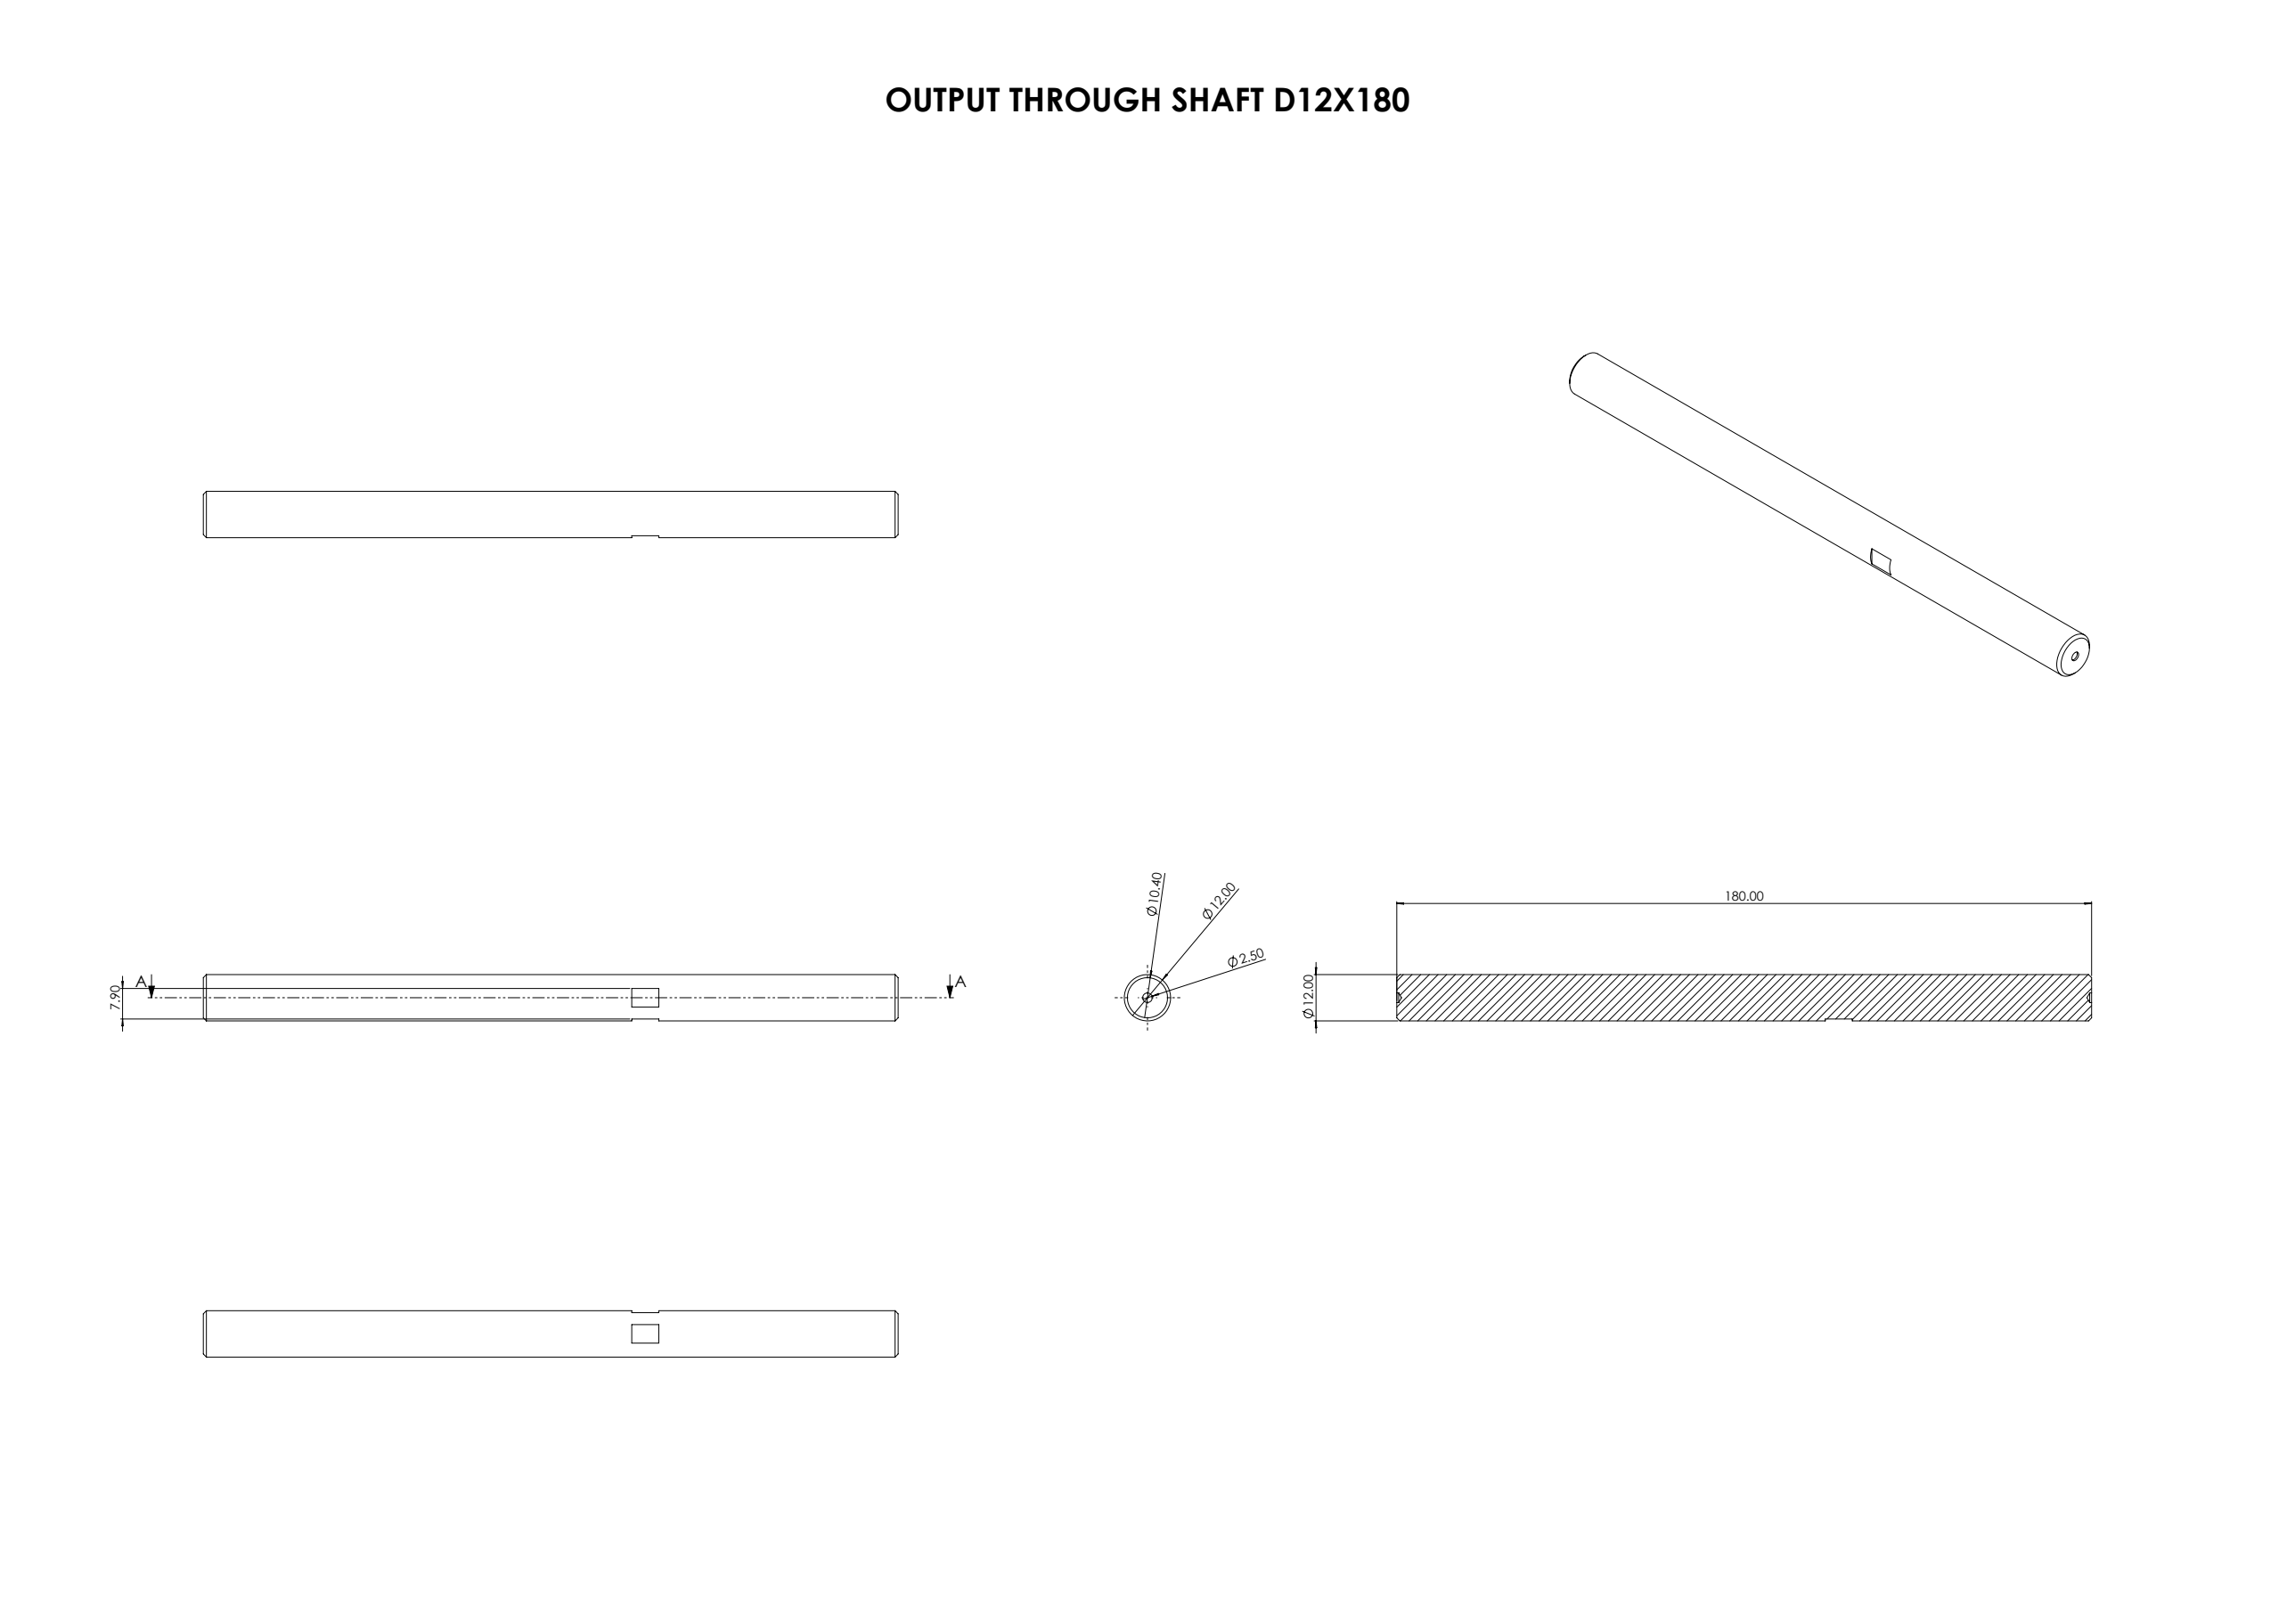
ISO-10303-21;
HEADER;
/* Generated by software containing ST-Developer
 * from STEP Tools, Inc. (www.steptools.com) 
 */

FILE_DESCRIPTION(
/* description */ (''),
/* implementation_level */ '2;1');

FILE_NAME(
/* name */ '05_Output_Through_Shaft_D12x180.step',
/* time_stamp */ '2026-10-11T09:12:28-07:00',
/* author */ (''),
/* organization */ (''),
/* preprocessor_version */ 'ST-DEVELOPER v20.2',
/* originating_system */ 'Autodesk Translation Framework v15.15.0.0',
/* authorisation */ '');

FILE_SCHEMA (('AUTOMOTIVE_DESIGN { 1 0 10303 214 3 1 1 }'));
ENDSEC;

DATA;
#10=MECHANICAL_DESIGN_GEOMETRIC_PRESENTATION_REPRESENTATION('',(#651),#23254);
#631=SHAPE_REPRESENTATION_RELATIONSHIP('SRR','None',#23304,#641);
#641=ADVANCED_BREP_SHAPE_REPRESENTATION('',(#661),#23248);
#651=STYLED_ITEM('',(#23462),#661);
#661=MANIFOLD_SOLID_BREP('Body1',#7029);
#739=CONICAL_SURFACE('',#7587,0.625,1.04746029293308);
#740=CONICAL_SURFACE('',#7594,1.25,1.04746029293308);
#741=CONICAL_SURFACE('',#7597,5.6,0.785398163397448);
#742=CONICAL_SURFACE('',#7601,5.6,0.785398163397448);
#811=FACE_BOUND('',#1692,.T.);
#812=FACE_BOUND('',#1695,.T.);
#813=FACE_BOUND('',#1698,.T.);
#940=PLANE('',#7575);
#941=PLANE('',#7578);
#942=PLANE('',#7581);
#943=PLANE('',#7582);
#944=PLANE('',#7584);
#945=PLANE('',#7585);
#946=PLANE('',#7595);
#947=PLANE('',#7603);
#1255=FACE_OUTER_BOUND('',#1681,.T.);
#1256=FACE_OUTER_BOUND('',#1682,.T.);
#1257=FACE_OUTER_BOUND('',#1683,.T.);
#1258=FACE_OUTER_BOUND('',#1684,.T.);
#1259=FACE_OUTER_BOUND('',#1685,.T.);
#1260=FACE_OUTER_BOUND('',#1686,.T.);
#1261=FACE_OUTER_BOUND('',#1687,.T.);
#1262=FACE_OUTER_BOUND('',#1688,.T.);
#1263=FACE_OUTER_BOUND('',#1689,.T.);
#1264=FACE_OUTER_BOUND('',#1690,.T.);
#1265=FACE_OUTER_BOUND('',#1691,.T.);
#1266=FACE_OUTER_BOUND('',#1693,.T.);
#1267=FACE_OUTER_BOUND('',#1694,.T.);
#1268=FACE_OUTER_BOUND('',#1696,.T.);
#1269=FACE_OUTER_BOUND('',#1697,.T.);
#1681=EDGE_LOOP('',(#5933,#5934,#5935));
#1682=EDGE_LOOP('',(#5936,#5937,#5938));
#1683=EDGE_LOOP('',(#5939,#5940,#5941,#5942));
#1684=EDGE_LOOP('',(#5943,#5944));
#1685=EDGE_LOOP('',(#5945,#5946,#5947,#5948));
#1686=EDGE_LOOP('',(#5949,#5950));
#1687=EDGE_LOOP('',(#5951,#5952,#5953));
#1688=EDGE_LOOP('',(#5954,#5955,#5956,#5957));
#1689=EDGE_LOOP('',(#5958,#5959,#5960,#5961));
#1690=EDGE_LOOP('',(#5962,#5963,#5964));
#1691=EDGE_LOOP('',(#5965));
#1692=EDGE_LOOP('',(#5966));
#1693=EDGE_LOOP('',(#5967,#5968,#5969,#5970));
#1694=EDGE_LOOP('',(#5971,#5972,#5973,#5974,#5975,#5976,#5977,#5978,#5979,
#5980,#5981,#5982));
#1695=EDGE_LOOP('',(#5983,#5984,#5985,#5986));
#1696=EDGE_LOOP('',(#5987,#5988,#5989,#5990));
#1697=EDGE_LOOP('',(#5991));
#1698=EDGE_LOOP('',(#5992));
#2009=LINE('',#21048,#2268);
#2010=LINE('',#21055,#2269);
#2011=LINE('',#21058,#2270);
#2012=LINE('',#21059,#2271);
#2013=LINE('',#21064,#2272);
#2014=LINE('',#21067,#2273);
#2015=LINE('',#21069,#2274);
#2016=LINE('',#21070,#2275);
#2017=LINE('',#21076,#2276);
#2018=LINE('',#21080,#2277);
#2019=LINE('',#21086,#2278);
#2020=LINE('',#21090,#2279);
#2021=LINE('',#21097,#2280);
#2022=LINE('',#21101,#2281);
#2023=LINE('',#21102,#2282);
#2024=LINE('',#21106,#2283);
#2268=VECTOR('',#8861,10.);
#2269=VECTOR('',#8868,10.);
#2270=VECTOR('',#8873,10.);
#2271=VECTOR('',#8874,10.);
#2272=VECTOR('',#8879,10.);
#2273=VECTOR('',#8882,10.);
#2274=VECTOR('',#8883,10.);
#2275=VECTOR('',#8884,10.);
#2276=VECTOR('',#8891,0.625);
#2277=VECTOR('',#8896,1.25);
#2278=VECTOR('',#8903,1.25);
#2279=VECTOR('',#8908,1.25);
#2280=VECTOR('',#8917,5.6);
#2281=VECTOR('',#8922,6.);
#2282=VECTOR('',#8923,6.);
#2283=VECTOR('',#8928,5.6);
#2586=CIRCLE('',#7576,6.);
#2587=CIRCLE('',#7577,6.);
#2588=CIRCLE('',#7579,6.);
#2589=CIRCLE('',#7580,6.);
#2590=CIRCLE('',#7583,6.);
#2591=CIRCLE('',#7586,6.);
#2592=CIRCLE('',#7588,1.25);
#2593=CIRCLE('',#7590,1.25);
#2594=CIRCLE('',#7592,1.25);
#2595=CIRCLE('',#7593,1.25);
#2596=CIRCLE('',#7596,5.2);
#2597=CIRCLE('',#7598,6.);
#2598=CIRCLE('',#7600,6.);
#2599=CIRCLE('',#7602,5.2);
#3184=VERTEX_POINT('',#21044);
#3185=VERTEX_POINT('',#21045);
#3186=VERTEX_POINT('',#21047);
#3187=VERTEX_POINT('',#21051);
#3188=VERTEX_POINT('',#21052);
#3189=VERTEX_POINT('',#21054);
#3190=VERTEX_POINT('',#21061);
#3191=VERTEX_POINT('',#21062);
#3192=VERTEX_POINT('',#21066);
#3193=VERTEX_POINT('',#21068);
#3194=VERTEX_POINT('',#21074);
#3195=VERTEX_POINT('',#21075);
#3196=VERTEX_POINT('',#21079);
#3197=VERTEX_POINT('',#21083);
#3198=VERTEX_POINT('',#21085);
#3199=VERTEX_POINT('',#21089);
#3200=VERTEX_POINT('',#21092);
#3201=VERTEX_POINT('',#21095);
#3202=VERTEX_POINT('',#21099);
#3203=VERTEX_POINT('',#21104);
#4142=EDGE_CURVE('',#3184,#3185,#2586,.T.);
#4143=EDGE_CURVE('',#3184,#3186,#2009,.T.);
#4144=EDGE_CURVE('',#3185,#3186,#2587,.T.);
#4145=EDGE_CURVE('',#3187,#3188,#2588,.T.);
#4146=EDGE_CURVE('',#3187,#3189,#2010,.T.);
#4147=EDGE_CURVE('',#3188,#3189,#2589,.T.);
#4148=EDGE_CURVE('',#3189,#3184,#2011,.T.);
#4149=EDGE_CURVE('',#3186,#3187,#2012,.T.);
#4150=EDGE_CURVE('',#3190,#3191,#2590,.T.);
#4151=EDGE_CURVE('',#3190,#3191,#2013,.T.);
#4152=EDGE_CURVE('',#3192,#3190,#2014,.T.);
#4153=EDGE_CURVE('',#3193,#3192,#2015,.T.);
#4154=EDGE_CURVE('',#3191,#3193,#2016,.T.);
#4155=EDGE_CURVE('',#3193,#3192,#2591,.T.);
#4156=EDGE_CURVE('',#3194,#3195,#2017,.T.);
#4157=EDGE_CURVE('',#3195,#3195,#2592,.T.);
#4158=EDGE_CURVE('',#3195,#3196,#2018,.T.);
#4159=EDGE_CURVE('',#3196,#3196,#2593,.T.);
#4160=EDGE_CURVE('',#3197,#3197,#2594,.T.);
#4161=EDGE_CURVE('',#3197,#3198,#2019,.T.);
#4162=EDGE_CURVE('',#3198,#3198,#2595,.T.);
#4163=EDGE_CURVE('',#3198,#3199,#2020,.T.);
#4164=EDGE_CURVE('',#3200,#3200,#2596,.T.);
#4165=EDGE_CURVE('',#3201,#3201,#2597,.T.);
#4166=EDGE_CURVE('',#3201,#3200,#2021,.T.);
#4167=EDGE_CURVE('',#3202,#3202,#2598,.T.);
#4168=EDGE_CURVE('',#3202,#3188,#2022,.T.);
#4169=EDGE_CURVE('',#3185,#3201,#2023,.T.);
#4170=EDGE_CURVE('',#3203,#3203,#2599,.T.);
#4171=EDGE_CURVE('',#3203,#3202,#2024,.T.);
#5933=ORIENTED_EDGE('',*,*,#4142,.F.);
#5934=ORIENTED_EDGE('',*,*,#4143,.T.);
#5935=ORIENTED_EDGE('',*,*,#4144,.F.);
#5936=ORIENTED_EDGE('',*,*,#4145,.F.);
#5937=ORIENTED_EDGE('',*,*,#4146,.T.);
#5938=ORIENTED_EDGE('',*,*,#4147,.F.);
#5939=ORIENTED_EDGE('',*,*,#4148,.F.);
#5940=ORIENTED_EDGE('',*,*,#4146,.F.);
#5941=ORIENTED_EDGE('',*,*,#4149,.F.);
#5942=ORIENTED_EDGE('',*,*,#4143,.F.);
#5943=ORIENTED_EDGE('',*,*,#4150,.F.);
#5944=ORIENTED_EDGE('',*,*,#4151,.T.);
#5945=ORIENTED_EDGE('',*,*,#4152,.F.);
#5946=ORIENTED_EDGE('',*,*,#4153,.F.);
#5947=ORIENTED_EDGE('',*,*,#4154,.F.);
#5948=ORIENTED_EDGE('',*,*,#4151,.F.);
#5949=ORIENTED_EDGE('',*,*,#4155,.F.);
#5950=ORIENTED_EDGE('',*,*,#4153,.T.);
#5951=ORIENTED_EDGE('',*,*,#4156,.T.);
#5952=ORIENTED_EDGE('',*,*,#4157,.T.);
#5953=ORIENTED_EDGE('',*,*,#4156,.F.);
#5954=ORIENTED_EDGE('',*,*,#4157,.F.);
#5955=ORIENTED_EDGE('',*,*,#4158,.T.);
#5956=ORIENTED_EDGE('',*,*,#4159,.F.);
#5957=ORIENTED_EDGE('',*,*,#4158,.F.);
#5958=ORIENTED_EDGE('',*,*,#4160,.F.);
#5959=ORIENTED_EDGE('',*,*,#4161,.T.);
#5960=ORIENTED_EDGE('',*,*,#4162,.T.);
#5961=ORIENTED_EDGE('',*,*,#4161,.F.);
#5962=ORIENTED_EDGE('',*,*,#4162,.F.);
#5963=ORIENTED_EDGE('',*,*,#4163,.T.);
#5964=ORIENTED_EDGE('',*,*,#4163,.F.);
#5965=ORIENTED_EDGE('',*,*,#4164,.F.);
#5966=ORIENTED_EDGE('',*,*,#4160,.T.);
#5967=ORIENTED_EDGE('',*,*,#4165,.F.);
#5968=ORIENTED_EDGE('',*,*,#4166,.T.);
#5969=ORIENTED_EDGE('',*,*,#4164,.T.);
#5970=ORIENTED_EDGE('',*,*,#4166,.F.);
#5971=ORIENTED_EDGE('',*,*,#4167,.F.);
#5972=ORIENTED_EDGE('',*,*,#4168,.T.);
#5973=ORIENTED_EDGE('',*,*,#4147,.T.);
#5974=ORIENTED_EDGE('',*,*,#4148,.T.);
#5975=ORIENTED_EDGE('',*,*,#4142,.T.);
#5976=ORIENTED_EDGE('',*,*,#4169,.T.);
#5977=ORIENTED_EDGE('',*,*,#4165,.T.);
#5978=ORIENTED_EDGE('',*,*,#4169,.F.);
#5979=ORIENTED_EDGE('',*,*,#4144,.T.);
#5980=ORIENTED_EDGE('',*,*,#4149,.T.);
#5981=ORIENTED_EDGE('',*,*,#4145,.T.);
#5982=ORIENTED_EDGE('',*,*,#4168,.F.);
#5983=ORIENTED_EDGE('',*,*,#4154,.T.);
#5984=ORIENTED_EDGE('',*,*,#4155,.T.);
#5985=ORIENTED_EDGE('',*,*,#4152,.T.);
#5986=ORIENTED_EDGE('',*,*,#4150,.T.);
#5987=ORIENTED_EDGE('',*,*,#4170,.F.);
#5988=ORIENTED_EDGE('',*,*,#4171,.T.);
#5989=ORIENTED_EDGE('',*,*,#4167,.T.);
#5990=ORIENTED_EDGE('',*,*,#4171,.F.);
#5991=ORIENTED_EDGE('',*,*,#4170,.T.);
#5992=ORIENTED_EDGE('',*,*,#4159,.T.);
#6602=CYLINDRICAL_SURFACE('',#7589,1.25);
#6603=CYLINDRICAL_SURFACE('',#7591,1.25);
#6604=CYLINDRICAL_SURFACE('',#7599,6.);
#6906=ADVANCED_FACE('',(#1255),#940,.F.);
#6907=ADVANCED_FACE('',(#1256),#941,.F.);
#6908=ADVANCED_FACE('',(#1257),#942,.F.);
#6909=ADVANCED_FACE('',(#1258),#943,.F.);
#6910=ADVANCED_FACE('',(#1259),#944,.F.);
#6911=ADVANCED_FACE('',(#1260),#945,.F.);
#6912=ADVANCED_FACE('',(#1261),#739,.F.);
#6913=ADVANCED_FACE('',(#1262),#6602,.F.);
#6914=ADVANCED_FACE('',(#1263),#6603,.F.);
#6915=ADVANCED_FACE('',(#1264),#740,.F.);
#6916=ADVANCED_FACE('',(#1265,#811),#946,.T.);
#6917=ADVANCED_FACE('',(#1266),#741,.T.);
#6918=ADVANCED_FACE('',(#1267,#812),#6604,.T.);
#6919=ADVANCED_FACE('',(#1268),#742,.T.);
#6920=ADVANCED_FACE('',(#1269,#813),#947,.T.);
#7029=CLOSED_SHELL('',(#6906,#6907,#6908,#6909,#6910,#6911,#6912,#6913,
#6914,#6915,#6916,#6917,#6918,#6919,#6920));
#7574=AXIS2_PLACEMENT_3D('',#21042,#8855,#8856);
#7575=AXIS2_PLACEMENT_3D('',#21043,#8857,#8858);
#7576=AXIS2_PLACEMENT_3D('',#21046,#8859,#8860);
#7577=AXIS2_PLACEMENT_3D('',#21049,#8862,#8863);
#7578=AXIS2_PLACEMENT_3D('',#21050,#8864,#8865);
#7579=AXIS2_PLACEMENT_3D('',#21053,#8866,#8867);
#7580=AXIS2_PLACEMENT_3D('',#21056,#8869,#8870);
#7581=AXIS2_PLACEMENT_3D('',#21057,#8871,#8872);
#7582=AXIS2_PLACEMENT_3D('',#21060,#8875,#8876);
#7583=AXIS2_PLACEMENT_3D('',#21063,#8877,#8878);
#7584=AXIS2_PLACEMENT_3D('',#21065,#8880,#8881);
#7585=AXIS2_PLACEMENT_3D('',#21071,#8885,#8886);
#7586=AXIS2_PLACEMENT_3D('',#21072,#8887,#8888);
#7587=AXIS2_PLACEMENT_3D('',#21073,#8889,#8890);
#7588=AXIS2_PLACEMENT_3D('',#21077,#8892,#8893);
#7589=AXIS2_PLACEMENT_3D('',#21078,#8894,#8895);
#7590=AXIS2_PLACEMENT_3D('',#21081,#8897,#8898);
#7591=AXIS2_PLACEMENT_3D('',#21082,#8899,#8900);
#7592=AXIS2_PLACEMENT_3D('',#21084,#8901,#8902);
#7593=AXIS2_PLACEMENT_3D('',#21087,#8904,#8905);
#7594=AXIS2_PLACEMENT_3D('',#21088,#8906,#8907);
#7595=AXIS2_PLACEMENT_3D('',#21091,#8909,#8910);
#7596=AXIS2_PLACEMENT_3D('',#21093,#8911,#8912);
#7597=AXIS2_PLACEMENT_3D('',#21094,#8913,#8914);
#7598=AXIS2_PLACEMENT_3D('',#21096,#8915,#8916);
#7599=AXIS2_PLACEMENT_3D('',#21098,#8918,#8919);
#7600=AXIS2_PLACEMENT_3D('',#21100,#8920,#8921);
#7601=AXIS2_PLACEMENT_3D('',#21103,#8924,#8925);
#7602=AXIS2_PLACEMENT_3D('',#21105,#8926,#8927);
#7603=AXIS2_PLACEMENT_3D('',#21107,#8929,#8930);
#8855=DIRECTION('axis',(0.,0.,1.));
#8856=DIRECTION('refdir',(1.,0.,0.));
#8857=DIRECTION('center_axis',(-1.,0.,0.));
#8858=DIRECTION('ref_axis',(0.,0.,1.));
#8859=DIRECTION('center_axis',(-1.,0.,0.));
#8860=DIRECTION('ref_axis',(0.,1.,0.));
#8861=DIRECTION('',(0.,0.,1.));
#8862=DIRECTION('center_axis',(-1.,0.,0.));
#8863=DIRECTION('ref_axis',(0.,1.,0.));
#8864=DIRECTION('center_axis',(1.,0.,0.));
#8865=DIRECTION('ref_axis',(0.,0.,-1.));
#8866=DIRECTION('center_axis',(1.,0.,0.));
#8867=DIRECTION('ref_axis',(0.,1.,0.));
#8868=DIRECTION('',(0.,0.,-1.));
#8869=DIRECTION('center_axis',(1.,0.,0.));
#8870=DIRECTION('ref_axis',(0.,1.,0.));
#8871=DIRECTION('center_axis',(0.,1.,0.));
#8872=DIRECTION('ref_axis',(0.,0.,1.));
#8873=DIRECTION('',(-1.,0.,0.));
#8874=DIRECTION('',(1.,0.,0.));
#8875=DIRECTION('center_axis',(-1.,0.,0.));
#8876=DIRECTION('ref_axis',(0.,-1.,0.));
#8877=DIRECTION('center_axis',(-1.,0.,0.));
#8878=DIRECTION('ref_axis',(0.,1.,0.));
#8879=DIRECTION('',(0.,1.,0.));
#8880=DIRECTION('center_axis',(0.,0.,-1.));
#8881=DIRECTION('ref_axis',(-1.,0.,0.));
#8882=DIRECTION('',(-1.,0.,0.));
#8883=DIRECTION('',(0.,-1.,0.));
#8884=DIRECTION('',(1.,0.,0.));
#8885=DIRECTION('center_axis',(1.,0.,0.));
#8886=DIRECTION('ref_axis',(0.,1.,0.));
#8887=DIRECTION('center_axis',(1.,0.,0.));
#8888=DIRECTION('ref_axis',(0.,1.,0.));
#8889=DIRECTION('center_axis',(1.,0.,0.));
#8890=DIRECTION('ref_axis',(0.,1.,0.));
#8891=DIRECTION('',(0.499772441725887,-0.866156744758906,-1.06073608502889E-16));
#8892=DIRECTION('center_axis',(1.,0.,0.));
#8893=DIRECTION('ref_axis',(0.,0.,-1.));
#8894=DIRECTION('center_axis',(1.,0.,0.));
#8895=DIRECTION('ref_axis',(0.,1.,0.));
#8896=DIRECTION('',(1.,0.,0.));
#8897=DIRECTION('center_axis',(-1.,0.,0.));
#8898=DIRECTION('ref_axis',(0.,1.,0.));
#8899=DIRECTION('center_axis',(1.,0.,0.));
#8900=DIRECTION('ref_axis',(0.,1.,0.));
#8901=DIRECTION('center_axis',(1.,0.,0.));
#8902=DIRECTION('ref_axis',(0.,1.,0.));
#8903=DIRECTION('',(1.,0.,0.));
#8904=DIRECTION('center_axis',(1.,0.,0.));
#8905=DIRECTION('ref_axis',(0.,0.,-1.));
#8906=DIRECTION('center_axis',(-1.,0.,0.));
#8907=DIRECTION('ref_axis',(0.,1.,0.));
#8908=DIRECTION('',(0.499772441725887,0.866156744758906,1.06073608502889E-16));
#8909=DIRECTION('center_axis',(-1.,0.,0.));
#8910=DIRECTION('ref_axis',(0.,0.,1.));
#8911=DIRECTION('center_axis',(1.,0.,0.));
#8912=DIRECTION('ref_axis',(0.,0.,-1.));
#8913=DIRECTION('center_axis',(1.,0.,0.));
#8914=DIRECTION('ref_axis',(0.,1.,0.));
#8915=DIRECTION('center_axis',(1.,0.,0.));
#8916=DIRECTION('ref_axis',(0.,0.,-1.));
#8917=DIRECTION('',(-0.707106781186548,0.707106781186547,8.65956056235493E-17));
#8918=DIRECTION('center_axis',(1.,0.,0.));
#8919=DIRECTION('ref_axis',(0.,1.,0.));
#8920=DIRECTION('center_axis',(1.,0.,0.));
#8921=DIRECTION('ref_axis',(0.,0.,-1.));
#8922=DIRECTION('',(-1.,0.,0.));
#8923=DIRECTION('',(-1.,0.,0.));
#8924=DIRECTION('center_axis',(-1.,0.,0.));
#8925=DIRECTION('ref_axis',(0.,1.,0.));
#8926=DIRECTION('center_axis',(1.,0.,0.));
#8927=DIRECTION('ref_axis',(0.,0.,-1.));
#8928=DIRECTION('',(-0.707106781186548,-0.707106781186547,-8.65956056235493E-17));
#8929=DIRECTION('center_axis',(1.,0.,0.));
#8930=DIRECTION('ref_axis',(0.,0.,-1.));
#21042=CARTESIAN_POINT('',(0.,0.,0.));
#21043=CARTESIAN_POINT('Origin',(21.,-6.,-7.));
#21044=CARTESIAN_POINT('',(21.,-5.5,-2.39791576165636));
#21045=CARTESIAN_POINT('',(21.,-6.,-7.34788079488412E-16));
#21046=CARTESIAN_POINT('Origin',(21.,0.,0.));
#21047=CARTESIAN_POINT('',(21.,-5.5,2.39791576165636));
#21048=CARTESIAN_POINT('',(21.,-5.5,7.));
#21049=CARTESIAN_POINT('Origin',(21.,0.,0.));
#21050=CARTESIAN_POINT('Origin',(28.,-6.,7.));
#21051=CARTESIAN_POINT('',(28.,-5.5,2.39791576165636));
#21052=CARTESIAN_POINT('',(28.,-6.,-7.34788079488412E-16));
#21053=CARTESIAN_POINT('Origin',(28.,0.,0.));
#21054=CARTESIAN_POINT('',(28.,-5.5,-2.39791576165636));
#21055=CARTESIAN_POINT('',(28.,-5.5,-7.));
#21056=CARTESIAN_POINT('Origin',(28.,0.,0.));
#21057=CARTESIAN_POINT('Origin',(24.5,-5.5,0.));
#21058=CARTESIAN_POINT('',(0.,-5.5,-2.39791576165636));
#21059=CARTESIAN_POINT('',(0.,-5.5,2.39791576165636));
#21060=CARTESIAN_POINT('Origin',(21.,7.,6.));
#21061=CARTESIAN_POINT('',(21.,-2.39791576165636,5.5));
#21062=CARTESIAN_POINT('',(21.,2.39791576165636,5.5));
#21063=CARTESIAN_POINT('Origin',(21.,0.,0.));
#21064=CARTESIAN_POINT('',(21.,7.,5.5));
#21065=CARTESIAN_POINT('Origin',(24.5,0.,5.5));
#21066=CARTESIAN_POINT('',(28.,-2.39791576165636,5.5));
#21067=CARTESIAN_POINT('',(0.,-2.39791576165636,5.5));
#21068=CARTESIAN_POINT('',(28.,2.39791576165636,5.5));
#21069=CARTESIAN_POINT('',(28.,-7.,5.5));
#21070=CARTESIAN_POINT('',(0.,2.39791576165636,5.5));
#21071=CARTESIAN_POINT('Origin',(28.,-7.,6.));
#21072=CARTESIAN_POINT('Origin',(28.,0.,0.));
#21073=CARTESIAN_POINT('Origin',(89.139375,0.,0.));
#21074=CARTESIAN_POINT('',(88.77875,0.,0.));
#21075=CARTESIAN_POINT('',(89.5,-1.25,-1.53080849893419E-16));
#21076=CARTESIAN_POINT('',(89.139375,-0.625,-7.65404249467096E-17));
#21077=CARTESIAN_POINT('Origin',(89.5,0.,0.));
#21078=CARTESIAN_POINT('Origin',(89.75,0.,0.));
#21079=CARTESIAN_POINT('',(90.,-1.25,-1.53080849893419E-16));
#21080=CARTESIAN_POINT('',(89.75,-1.25,-1.53080849893419E-16));
#21081=CARTESIAN_POINT('Origin',(90.,0.,0.));
#21082=CARTESIAN_POINT('Origin',(-89.75,0.,0.));
#21083=CARTESIAN_POINT('',(-90.,-1.25,-1.53080849893419E-16));
#21084=CARTESIAN_POINT('Origin',(-90.,0.,0.));
#21085=CARTESIAN_POINT('',(-89.5,-1.25,-1.53080849893419E-16));
#21086=CARTESIAN_POINT('',(-89.75,-1.25,-1.53080849893419E-16));
#21087=CARTESIAN_POINT('Origin',(-89.5,0.,0.));
#21088=CARTESIAN_POINT('Origin',(-89.5,0.,0.));
#21089=CARTESIAN_POINT('',(-88.77875,0.,0.));
#21090=CARTESIAN_POINT('',(-89.5,-1.25,-1.53080849893419E-16));
#21091=CARTESIAN_POINT('Origin',(-90.,5.2,0.));
#21092=CARTESIAN_POINT('',(-90.,-5.2,-6.36816335556624E-16));
#21093=CARTESIAN_POINT('Origin',(-90.,0.,0.));
#21094=CARTESIAN_POINT('Origin',(-89.6,0.,0.));
#21095=CARTESIAN_POINT('',(-89.2,-6.,-7.34788079488411E-16));
#21096=CARTESIAN_POINT('Origin',(-89.2,0.,0.));
#21097=CARTESIAN_POINT('',(-89.6,-5.6,-6.85802207522518E-16));
#21098=CARTESIAN_POINT('Origin',(0.,0.,0.));
#21099=CARTESIAN_POINT('',(89.2,-6.,-7.34788079488412E-16));
#21100=CARTESIAN_POINT('Origin',(89.2,0.,0.));
#21101=CARTESIAN_POINT('',(0.,-6.,-7.34788079488412E-16));
#21102=CARTESIAN_POINT('',(0.,-6.,-7.34788079488412E-16));
#21103=CARTESIAN_POINT('Origin',(89.6,0.,0.));
#21104=CARTESIAN_POINT('',(90.,-5.2,-6.36816335556624E-16));
#21105=CARTESIAN_POINT('Origin',(90.,0.,0.));
#21106=CARTESIAN_POINT('',(89.6,-5.6,-6.85802207522518E-16));
#21107=CARTESIAN_POINT('Origin',(90.,0.,0.));
#23236=UNCERTAINTY_MEASURE_WITH_UNIT(LENGTH_MEASURE(0.01),#23255,
'DISTANCE_ACCURACY_VALUE',
'Maximum model space distance between geometric entities at asserted c
onnectivities');
#23242=UNCERTAINTY_MEASURE_WITH_UNIT(LENGTH_MEASURE(0.01),#23255,
'DISTANCE_ACCURACY_VALUE',
'Maximum model space distance between geometric entities at asserted c
onnectivities');
#23248=(
GEOMETRIC_REPRESENTATION_CONTEXT(3)
GLOBAL_UNCERTAINTY_ASSIGNED_CONTEXT((#23236))
GLOBAL_UNIT_ASSIGNED_CONTEXT((#23255,#23257,#23258))
REPRESENTATION_CONTEXT('','3D')
);
#23254=(
GEOMETRIC_REPRESENTATION_CONTEXT(3)
GLOBAL_UNCERTAINTY_ASSIGNED_CONTEXT((#23242))
GLOBAL_UNIT_ASSIGNED_CONTEXT((#23255,#23257,#23258))
REPRESENTATION_CONTEXT('','3D')
);
#23255=(
LENGTH_UNIT()
NAMED_UNIT(*)
SI_UNIT(.MILLI.,.METRE.)
);
#23257=(
NAMED_UNIT(*)
PLANE_ANGLE_UNIT()
SI_UNIT($,.RADIAN.)
);
#23258=(
NAMED_UNIT(*)
SI_UNIT($,.STERADIAN.)
SOLID_ANGLE_UNIT()
);
#23264=SHAPE_DEFINITION_REPRESENTATION(#23275,#23304);
#23275=PRODUCT_DEFINITION_SHAPE('',$,#23316);
#23304=SHAPE_REPRESENTATION('',(#7574),#23248);
#23310=PRODUCT_DEFINITION_CONTEXT('part definition',#23345,'design');
#23316=PRODUCT_DEFINITION('2026-10-11-09-11-52-446',
'05_Output_Through_Shaft_D12x180',#23327,#23310);
#23327=PRODUCT_DEFINITION_FORMATION('',$,#23352);
#23345=APPLICATION_CONTEXT(
'Core Data for Automotive Mechanical Design Process');
#23346=PRODUCT_CONTEXT('part definition',#23345,'mechanical');
#23352=PRODUCT('2026-10-11-09-11-52-446',
'05_Output_Through_Shaft_D12x180',$,(#23346));
#23456=COLOUR_RGB('Grey',0.48,0.52,0.57);
#23457=FILL_AREA_STYLE_COLOUR('',#23456);
#23458=FILL_AREA_STYLE('',(#23457));
#23459=SURFACE_STYLE_FILL_AREA(#23458);
#23460=SURFACE_SIDE_STYLE('',(#23459));
#23461=SURFACE_STYLE_USAGE(.BOTH.,#23460);
#23462=PRESENTATION_STYLE_ASSIGNMENT((#23461));
ENDSEC;
END-ISO-10303-21;
